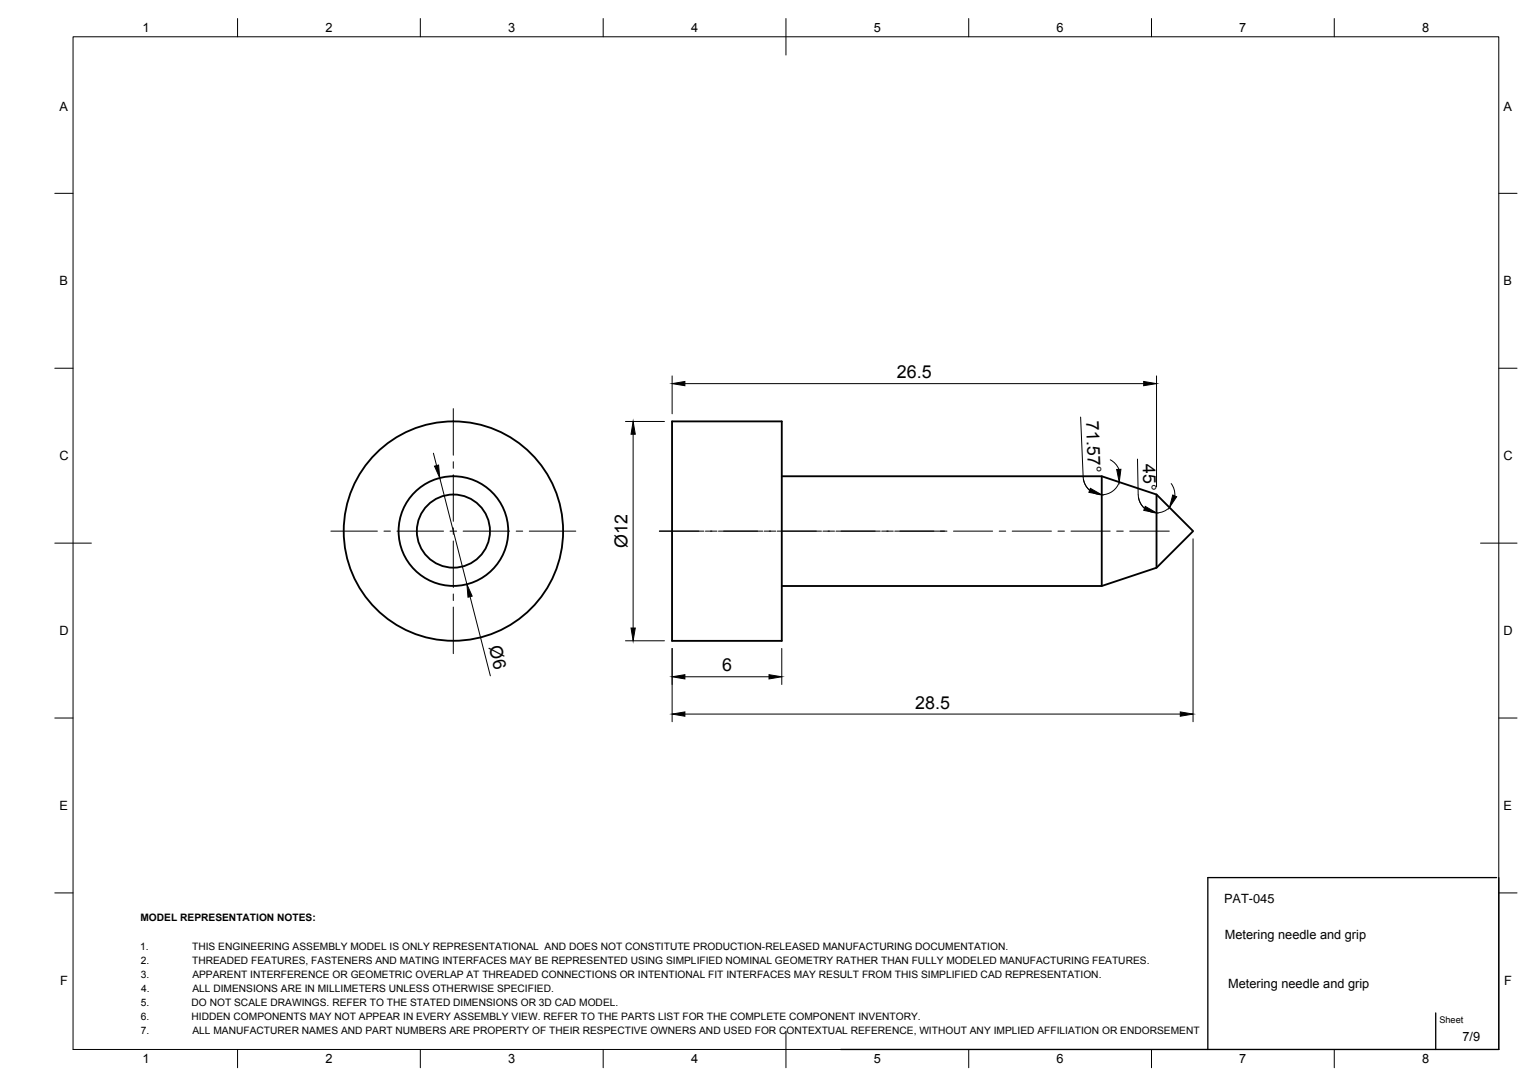
ISO-10303-21;
HEADER;
/* Generated by software containing ST-Developer
 * from STEP Tools, Inc. (www.steptools.com) 
 */

FILE_DESCRIPTION(
/* description */ ('Gauge isolation and snubber set'),
/* implementation_level */ '2;1');

FILE_NAME(
/* name */ 'Metering needle and grip.step',
/* time_stamp */ '2026-10-29T16:58:15-07:00',
/* author */ (''),
/* organization */ (''),
/* preprocessor_version */ 'ST-DEVELOPER v20.2',
/* originating_system */ 'Autodesk Translation Framework v15.17.0.0',
/* authorisation */ '');

FILE_SCHEMA (('AUTOMOTIVE_DESIGN { 1 0 10303 214 3 1 1 }'));
ENDSEC;

DATA;
#10=MECHANICAL_DESIGN_GEOMETRIC_PRESENTATION_REPRESENTATION('',(#96),#4043);
#72=CONICAL_SURFACE('',#2492,0.1,0.78539816339745);
#73=CONICAL_SURFACE('',#2494,0.25,0.321750554396641);
#80=SHAPE_REPRESENTATION_RELATIONSHIP('SRR','None',#4087,#88);
#88=ADVANCED_BREP_SHAPE_REPRESENTATION('',(#106),#4039);
#96=STYLED_ITEM('',(#4204),#106);
#106=MANIFOLD_SOLID_BREP('Body1',#2213);
#150=FACE_BOUND('',#497,.T.);
#218=PLANE('',#2498);
#219=PLANE('',#2502);
#331=FACE_OUTER_BOUND('',#493,.T.);
#332=FACE_OUTER_BOUND('',#494,.T.);
#333=FACE_OUTER_BOUND('',#495,.T.);
#334=FACE_OUTER_BOUND('',#496,.T.);
#335=FACE_OUTER_BOUND('',#498,.T.);
#336=FACE_OUTER_BOUND('',#499,.T.);
#493=EDGE_LOOP('',(#1925,#1926,#1927));
#494=EDGE_LOOP('',(#1928,#1929,#1930,#1931));
#495=EDGE_LOOP('',(#1932,#1933,#1934,#1935));
#496=EDGE_LOOP('',(#1936));
#497=EDGE_LOOP('',(#1937));
#498=EDGE_LOOP('',(#1938,#1939,#1940,#1941));
#499=EDGE_LOOP('',(#1942));
#617=CIRCLE('',#2493,0.2);
#618=CIRCLE('',#2495,0.3);
#619=CIRCLE('',#2497,0.3);
#620=CIRCLE('',#2499,0.6);
#621=CIRCLE('',#2501,0.6);
#768=LINE('',#3865,#939);
#769=LINE('',#3869,#940);
#770=LINE('',#3873,#941);
#771=LINE('',#3880,#942);
#939=VECTOR('',#3065,0.1);
#940=VECTOR('',#3070,0.25);
#941=VECTOR('',#3075,0.3);
#942=VECTOR('',#3084,0.6);
#1130=VERTEX_POINT('',#3862);
#1131=VERTEX_POINT('',#3864);
#1132=VERTEX_POINT('',#3867);
#1133=VERTEX_POINT('',#3871);
#1134=VERTEX_POINT('',#3875);
#1135=VERTEX_POINT('',#3878);
#1401=EDGE_CURVE('',#1130,#1130,#617,.T.);
#1402=EDGE_CURVE('',#1130,#1131,#768,.T.);
#1403=EDGE_CURVE('',#1132,#1132,#618,.T.);
#1404=EDGE_CURVE('',#1132,#1130,#769,.T.);
#1405=EDGE_CURVE('',#1133,#1133,#619,.T.);
#1406=EDGE_CURVE('',#1133,#1132,#770,.T.);
#1407=EDGE_CURVE('',#1134,#1134,#620,.T.);
#1408=EDGE_CURVE('',#1135,#1135,#621,.T.);
#1409=EDGE_CURVE('',#1135,#1134,#771,.T.);
#1925=ORIENTED_EDGE('',*,*,#1401,.F.);
#1926=ORIENTED_EDGE('',*,*,#1402,.T.);
#1927=ORIENTED_EDGE('',*,*,#1402,.F.);
#1928=ORIENTED_EDGE('',*,*,#1403,.F.);
#1929=ORIENTED_EDGE('',*,*,#1404,.T.);
#1930=ORIENTED_EDGE('',*,*,#1401,.T.);
#1931=ORIENTED_EDGE('',*,*,#1404,.F.);
#1932=ORIENTED_EDGE('',*,*,#1405,.F.);
#1933=ORIENTED_EDGE('',*,*,#1406,.T.);
#1934=ORIENTED_EDGE('',*,*,#1403,.T.);
#1935=ORIENTED_EDGE('',*,*,#1406,.F.);
#1936=ORIENTED_EDGE('',*,*,#1407,.F.);
#1937=ORIENTED_EDGE('',*,*,#1405,.T.);
#1938=ORIENTED_EDGE('',*,*,#1408,.F.);
#1939=ORIENTED_EDGE('',*,*,#1409,.T.);
#1940=ORIENTED_EDGE('',*,*,#1407,.T.);
#1941=ORIENTED_EDGE('',*,*,#1409,.F.);
#1942=ORIENTED_EDGE('',*,*,#1408,.T.);
#2079=CYLINDRICAL_SURFACE('',#2496,0.3);
#2080=CYLINDRICAL_SURFACE('',#2500,0.6);
#2175=ADVANCED_FACE('',(#331),#72,.T.);
#2176=ADVANCED_FACE('',(#332),#73,.T.);
#2177=ADVANCED_FACE('',(#333),#2079,.T.);
#2178=ADVANCED_FACE('',(#334,#150),#218,.T.);
#2179=ADVANCED_FACE('',(#335),#2080,.T.);
#2180=ADVANCED_FACE('',(#336),#219,.T.);
#2213=CLOSED_SHELL('',(#2175,#2176,#2177,#2178,#2179,#2180));
#2491=AXIS2_PLACEMENT_3D('',#3860,#3059,#3060);
#2492=AXIS2_PLACEMENT_3D('',#3861,#3061,#3062);
#2493=AXIS2_PLACEMENT_3D('',#3863,#3063,#3064);
#2494=AXIS2_PLACEMENT_3D('',#3866,#3066,#3067);
#2495=AXIS2_PLACEMENT_3D('',#3868,#3068,#3069);
#2496=AXIS2_PLACEMENT_3D('',#3870,#3071,#3072);
#2497=AXIS2_PLACEMENT_3D('',#3872,#3073,#3074);
#2498=AXIS2_PLACEMENT_3D('',#3874,#3076,#3077);
#2499=AXIS2_PLACEMENT_3D('',#3876,#3078,#3079);
#2500=AXIS2_PLACEMENT_3D('',#3877,#3080,#3081);
#2501=AXIS2_PLACEMENT_3D('',#3879,#3082,#3083);
#2502=AXIS2_PLACEMENT_3D('',#3881,#3085,#3086);
#3059=DIRECTION('axis',(0.,0.,1.));
#3060=DIRECTION('refdir',(1.,0.,0.));
#3061=DIRECTION('center_axis',(0.,0.,1.));
#3062=DIRECTION('ref_axis',(1.,0.,0.));
#3063=DIRECTION('center_axis',(0.,0.,1.));
#3064=DIRECTION('ref_axis',(1.,0.,0.));
#3065=DIRECTION('',(0.707106781186549,8.65956056235495E-17,-0.707106781186546));
#3066=DIRECTION('center_axis',(0.,0.,1.));
#3067=DIRECTION('ref_axis',(1.,0.,0.));
#3068=DIRECTION('center_axis',(0.,0.,1.));
#3069=DIRECTION('ref_axis',(1.,0.,0.));
#3070=DIRECTION('',(0.316227766016837,3.87267321454038E-17,-0.948683298050514));
#3071=DIRECTION('center_axis',(0.,0.,1.));
#3072=DIRECTION('ref_axis',(1.,0.,0.));
#3073=DIRECTION('center_axis',(0.,0.,1.));
#3074=DIRECTION('ref_axis',(1.,0.,0.));
#3075=DIRECTION('',(0.,0.,-1.));
#3076=DIRECTION('center_axis',(0.,0.,-1.));
#3077=DIRECTION('ref_axis',(-1.,0.,0.));
#3078=DIRECTION('center_axis',(0.,0.,1.));
#3079=DIRECTION('ref_axis',(1.,0.,0.));
#3080=DIRECTION('center_axis',(0.,0.,1.));
#3081=DIRECTION('ref_axis',(1.,0.,0.));
#3082=DIRECTION('center_axis',(0.,0.,1.));
#3083=DIRECTION('ref_axis',(1.,0.,0.));
#3084=DIRECTION('',(0.,0.,-1.));
#3085=DIRECTION('center_axis',(0.,0.,1.));
#3086=DIRECTION('ref_axis',(1.,0.,0.));
#3860=CARTESIAN_POINT('',(0.,0.,0.));
#3861=CARTESIAN_POINT('Origin',(0.,0.8,8.15));
#3862=CARTESIAN_POINT('',(-0.2,0.8,8.25));
#3863=CARTESIAN_POINT('Origin',(0.,0.8,8.25));
#3864=CARTESIAN_POINT('',(0.,0.8,8.05));
#3865=CARTESIAN_POINT('',(-0.1,0.8,8.15));
#3866=CARTESIAN_POINT('Origin',(0.,0.8,8.4));
#3867=CARTESIAN_POINT('',(-0.3,0.8,8.55));
#3868=CARTESIAN_POINT('Origin',(0.,0.8,8.55));
#3869=CARTESIAN_POINT('',(-0.25,0.8,8.4));
#3870=CARTESIAN_POINT('Origin',(0.,0.8,9.425));
#3871=CARTESIAN_POINT('',(-0.3,0.8,10.3));
#3872=CARTESIAN_POINT('Origin',(0.,0.8,10.3));
#3873=CARTESIAN_POINT('',(-0.3,0.8,9.425));
#3874=CARTESIAN_POINT('Origin',(0.6,0.8,10.3));
#3875=CARTESIAN_POINT('',(-0.6,0.8,10.3));
#3876=CARTESIAN_POINT('Origin',(0.,0.8,10.3));
#3877=CARTESIAN_POINT('Origin',(0.,0.8,10.6));
#3878=CARTESIAN_POINT('',(-0.6,0.8,10.9));
#3879=CARTESIAN_POINT('Origin',(0.,0.8,10.9));
#3880=CARTESIAN_POINT('',(-0.6,0.8,10.6));
#3881=CARTESIAN_POINT('Origin',(0.,0.8,10.9));
#4028=UNCERTAINTY_MEASURE_WITH_UNIT(LENGTH_MEASURE(0.001),#4044,
'DISTANCE_ACCURACY_VALUE',
'Maximum model space distance between geometric entities at asserted c
onnectivities');
#4032=UNCERTAINTY_MEASURE_WITH_UNIT(LENGTH_MEASURE(0.001),#4044,
'DISTANCE_ACCURACY_VALUE',
'Maximum model space distance between geometric entities at asserted c
onnectivities');
#4039=(
GEOMETRIC_REPRESENTATION_CONTEXT(3)
GLOBAL_UNCERTAINTY_ASSIGNED_CONTEXT((#4028))
GLOBAL_UNIT_ASSIGNED_CONTEXT((#4044,#4046,#4047))
REPRESENTATION_CONTEXT('','3D')
);
#4043=(
GEOMETRIC_REPRESENTATION_CONTEXT(3)
GLOBAL_UNCERTAINTY_ASSIGNED_CONTEXT((#4032))
GLOBAL_UNIT_ASSIGNED_CONTEXT((#4044,#4046,#4047))
REPRESENTATION_CONTEXT('','3D')
);
#4044=(
LENGTH_UNIT()
NAMED_UNIT(*)
SI_UNIT(.CENTI.,.METRE.)
);
#4046=(
NAMED_UNIT(*)
PLANE_ANGLE_UNIT()
SI_UNIT($,.RADIAN.)
);
#4047=(
NAMED_UNIT(*)
SI_UNIT($,.STERADIAN.)
SOLID_ANGLE_UNIT()
);
#4054=SHAPE_DEFINITION_REPRESENTATION(#4064,#4087);
#4064=PRODUCT_DEFINITION_SHAPE('',$,#4098);
#4087=SHAPE_REPRESENTATION('',(#2491),#4039);
#4091=PRODUCT_DEFINITION_CONTEXT('part definition',#4123,'design');
#4098=PRODUCT_DEFINITION('Metering needle and grip',
'Metering needle and grip',#4108,#4091);
#4108=PRODUCT_DEFINITION_FORMATION('',$,#4131);
#4123=APPLICATION_CONTEXT(
'Core Data for Automotive Mechanical Design Process');
#4124=PRODUCT_CONTEXT('part definition',#4123,'mechanical');
#4131=PRODUCT('Metering needle and grip','Metering needle and grip',
'Metering needle and grip',(#4124));
#4198=COLOUR_RGB('Black',0.12,0.14,0.17);
#4199=FILL_AREA_STYLE_COLOUR('',#4198);
#4200=FILL_AREA_STYLE('',(#4199));
#4201=SURFACE_STYLE_FILL_AREA(#4200);
#4202=SURFACE_SIDE_STYLE('',(#4201));
#4203=SURFACE_STYLE_USAGE(.BOTH.,#4202);
#4204=PRESENTATION_STYLE_ASSIGNMENT((#4203));
ENDSEC;
END-ISO-10303-21;
